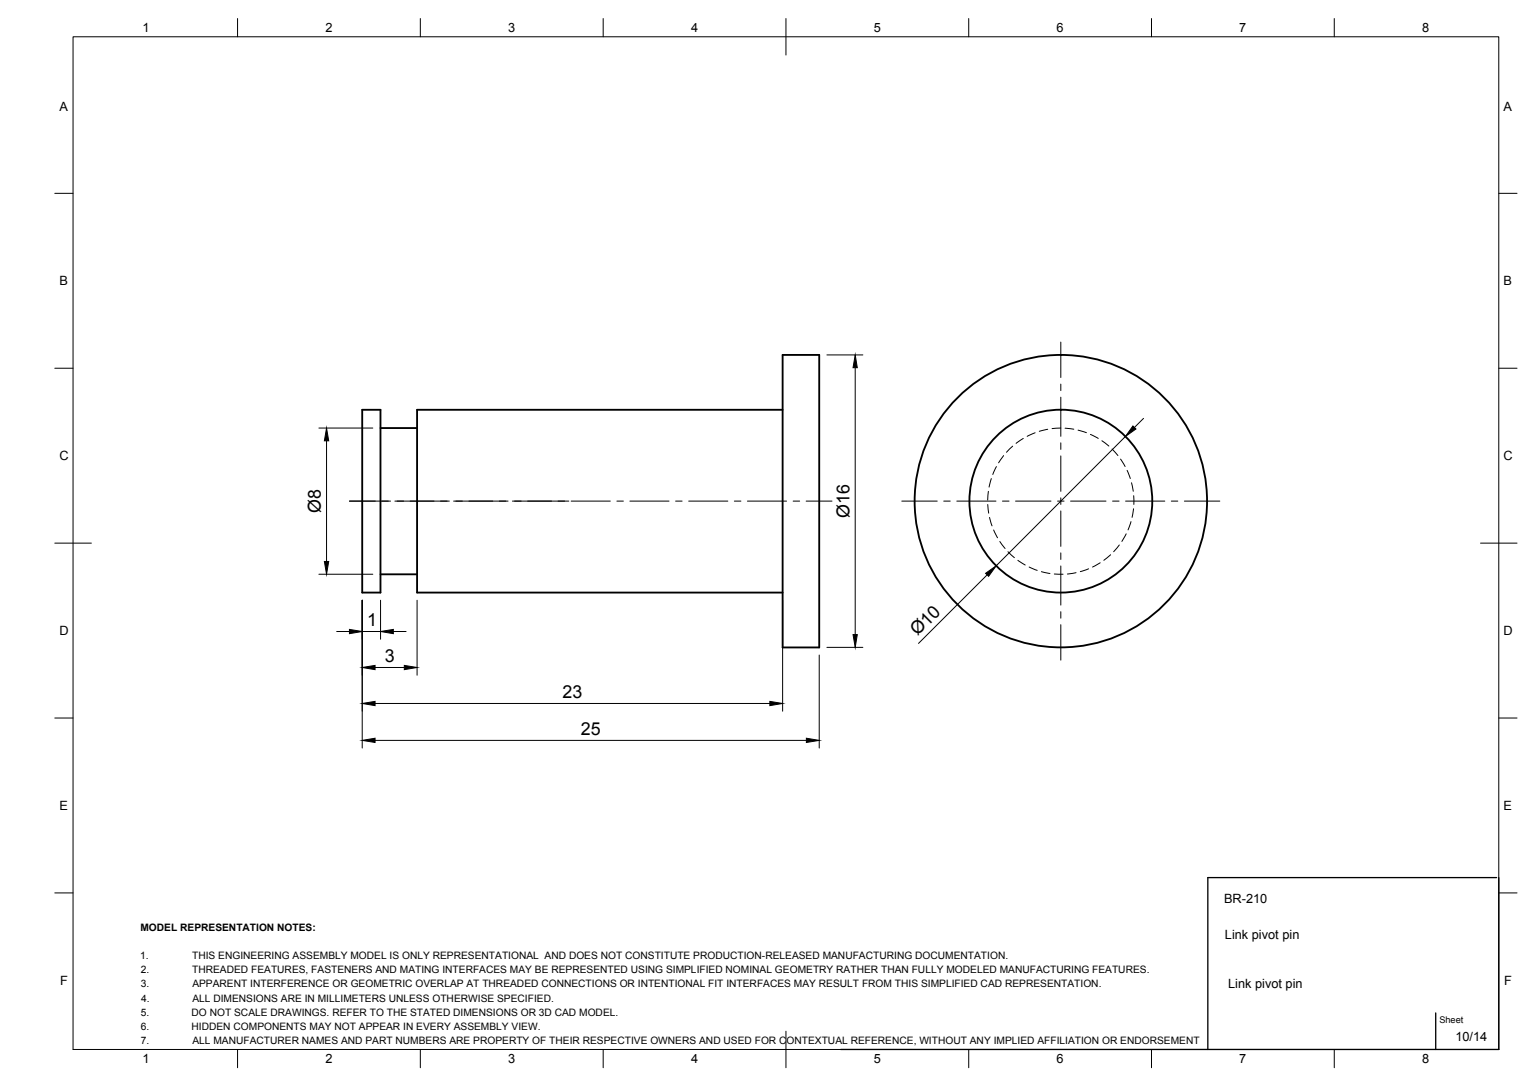
ISO-10303-21;
HEADER;
/* Generated by software containing ST-Developer
 * from STEP Tools, Inc. (www.steptools.com) 
 */

FILE_DESCRIPTION(
/* description */ ('Independent 1:2 reduction pantograph. 120 mm parallelogram sides; fix
ed fulcrum on the extension of a 240 mm link. Drawing point halfway al
ong its link, so its XY displacement is one half of the tracing point.
 Replaceable pivot bushes and retained pins. Calibration and productio
n accuracy unassigned.'),
/* implementation_level */ '2;1');

FILE_NAME(
/* name */ 'Link pivot pin.step',
/* time_stamp */ '2026-11-07T22:11:57-08:00',
/* author */ (''),
/* organization */ (''),
/* preprocessor_version */ 'ST-DEVELOPER v20.2',
/* originating_system */ 'Autodesk Translation Framework v15.17.0.0',
/* authorisation */ '');

FILE_SCHEMA (('AUTOMOTIVE_DESIGN { 1 0 10303 214 3 1 1 }'));
ENDSEC;

DATA;
#10=MECHANICAL_DESIGN_GEOMETRIC_PRESENTATION_REPRESENTATION('',(#195),#2926);
#169=SHAPE_REPRESENTATION_RELATIONSHIP('SRR','None',#3006,#182);
#182=ADVANCED_BREP_SHAPE_REPRESENTATION('',(#208),#2922);
#195=STYLED_ITEM('',(#3075),#208);
#208=MANIFOLD_SOLID_BREP('Body1',#1550);
#253=FACE_BOUND('',#510,.T.);
#254=FACE_BOUND('',#512,.T.);
#255=FACE_BOUND('',#515,.T.);
#293=PLANE('',#1852);
#294=PLANE('',#1854);
#295=PLANE('',#1858);
#296=PLANE('',#1863);
#297=PLANE('',#1865);
#375=FACE_OUTER_BOUND('',#508,.T.);
#376=FACE_OUTER_BOUND('',#509,.T.);
#377=FACE_OUTER_BOUND('',#511,.T.);
#378=FACE_OUTER_BOUND('',#513,.T.);
#379=FACE_OUTER_BOUND('',#514,.T.);
#380=FACE_OUTER_BOUND('',#516,.T.);
#381=FACE_OUTER_BOUND('',#517,.T.);
#382=FACE_OUTER_BOUND('',#518,.T.);
#383=FACE_OUTER_BOUND('',#519,.T.);
#508=EDGE_LOOP('',(#1337,#1338,#1339,#1340));
#509=EDGE_LOOP('',(#1341));
#510=EDGE_LOOP('',(#1342));
#511=EDGE_LOOP('',(#1343));
#512=EDGE_LOOP('',(#1344));
#513=EDGE_LOOP('',(#1345,#1346,#1347,#1348));
#514=EDGE_LOOP('',(#1349));
#515=EDGE_LOOP('',(#1350));
#516=EDGE_LOOP('',(#1351,#1352,#1353,#1354));
#517=EDGE_LOOP('',(#1355));
#518=EDGE_LOOP('',(#1356,#1357,#1358,#1359));
#519=EDGE_LOOP('',(#1360));
#600=LINE('',#2782,#681);
#601=LINE('',#2793,#682);
#602=LINE('',#2801,#683);
#603=LINE('',#2805,#684);
#681=VECTOR('',#2300,4.);
#682=VECTOR('',#2315,5.);
#683=VECTOR('',#2324,8.);
#684=VECTOR('',#2331,5.);
#767=CIRCLE('',#1850,4.);
#768=CIRCLE('',#1851,4.);
#769=CIRCLE('',#1853,5.);
#770=CIRCLE('',#1855,5.);
#771=CIRCLE('',#1857,5.);
#772=CIRCLE('',#1859,8.);
#773=CIRCLE('',#1860,5.);
#774=CIRCLE('',#1862,8.);
#875=VERTEX_POINT('',#2779);
#876=VERTEX_POINT('',#2781);
#877=VERTEX_POINT('',#2785);
#878=VERTEX_POINT('',#2788);
#879=VERTEX_POINT('',#2791);
#880=VERTEX_POINT('',#2795);
#881=VERTEX_POINT('',#2797);
#882=VERTEX_POINT('',#2800);
#1033=EDGE_CURVE('',#875,#875,#767,.T.);
#1034=EDGE_CURVE('',#875,#876,#600,.T.);
#1035=EDGE_CURVE('',#876,#876,#768,.T.);
#1036=EDGE_CURVE('',#877,#877,#769,.T.);
#1037=EDGE_CURVE('',#878,#878,#770,.T.);
#1038=EDGE_CURVE('',#879,#879,#771,.T.);
#1039=EDGE_CURVE('',#879,#878,#601,.T.);
#1040=EDGE_CURVE('',#880,#880,#772,.T.);
#1041=EDGE_CURVE('',#881,#881,#773,.T.);
#1042=EDGE_CURVE('',#880,#882,#602,.T.);
#1043=EDGE_CURVE('',#882,#882,#774,.T.);
#1044=EDGE_CURVE('',#877,#881,#603,.T.);
#1337=ORIENTED_EDGE('',*,*,#1033,.T.);
#1338=ORIENTED_EDGE('',*,*,#1034,.T.);
#1339=ORIENTED_EDGE('',*,*,#1035,.F.);
#1340=ORIENTED_EDGE('',*,*,#1034,.F.);
#1341=ORIENTED_EDGE('',*,*,#1036,.F.);
#1342=ORIENTED_EDGE('',*,*,#1033,.F.);
#1343=ORIENTED_EDGE('',*,*,#1037,.F.);
#1344=ORIENTED_EDGE('',*,*,#1035,.T.);
#1345=ORIENTED_EDGE('',*,*,#1038,.F.);
#1346=ORIENTED_EDGE('',*,*,#1039,.T.);
#1347=ORIENTED_EDGE('',*,*,#1037,.T.);
#1348=ORIENTED_EDGE('',*,*,#1039,.F.);
#1349=ORIENTED_EDGE('',*,*,#1040,.T.);
#1350=ORIENTED_EDGE('',*,*,#1041,.F.);
#1351=ORIENTED_EDGE('',*,*,#1040,.F.);
#1352=ORIENTED_EDGE('',*,*,#1042,.T.);
#1353=ORIENTED_EDGE('',*,*,#1043,.T.);
#1354=ORIENTED_EDGE('',*,*,#1042,.F.);
#1355=ORIENTED_EDGE('',*,*,#1043,.F.);
#1356=ORIENTED_EDGE('',*,*,#1036,.T.);
#1357=ORIENTED_EDGE('',*,*,#1044,.T.);
#1358=ORIENTED_EDGE('',*,*,#1041,.T.);
#1359=ORIENTED_EDGE('',*,*,#1044,.F.);
#1360=ORIENTED_EDGE('',*,*,#1038,.T.);
#1440=CYLINDRICAL_SURFACE('',#1849,4.);
#1441=CYLINDRICAL_SURFACE('',#1856,5.);
#1442=CYLINDRICAL_SURFACE('',#1861,8.);
#1443=CYLINDRICAL_SURFACE('',#1864,5.);
#1519=ADVANCED_FACE('',(#375),#1440,.T.);
#1520=ADVANCED_FACE('',(#376,#253),#293,.F.);
#1521=ADVANCED_FACE('',(#377,#254),#294,.F.);
#1522=ADVANCED_FACE('',(#378),#1441,.T.);
#1523=ADVANCED_FACE('',(#379,#255),#295,.T.);
#1524=ADVANCED_FACE('',(#380),#1442,.T.);
#1525=ADVANCED_FACE('',(#381),#296,.F.);
#1526=ADVANCED_FACE('',(#382),#1443,.T.);
#1527=ADVANCED_FACE('',(#383),#297,.T.);
#1550=CLOSED_SHELL('',(#1519,#1520,#1521,#1522,#1523,#1524,#1525,#1526,
#1527));
#1848=AXIS2_PLACEMENT_3D('',#2777,#2294,#2295);
#1849=AXIS2_PLACEMENT_3D('',#2778,#2296,#2297);
#1850=AXIS2_PLACEMENT_3D('',#2780,#2298,#2299);
#1851=AXIS2_PLACEMENT_3D('',#2783,#2301,#2302);
#1852=AXIS2_PLACEMENT_3D('',#2784,#2303,#2304);
#1853=AXIS2_PLACEMENT_3D('',#2786,#2305,#2306);
#1854=AXIS2_PLACEMENT_3D('',#2787,#2307,#2308);
#1855=AXIS2_PLACEMENT_3D('',#2789,#2309,#2310);
#1856=AXIS2_PLACEMENT_3D('',#2790,#2311,#2312);
#1857=AXIS2_PLACEMENT_3D('',#2792,#2313,#2314);
#1858=AXIS2_PLACEMENT_3D('',#2794,#2316,#2317);
#1859=AXIS2_PLACEMENT_3D('',#2796,#2318,#2319);
#1860=AXIS2_PLACEMENT_3D('',#2798,#2320,#2321);
#1861=AXIS2_PLACEMENT_3D('',#2799,#2322,#2323);
#1862=AXIS2_PLACEMENT_3D('',#2802,#2325,#2326);
#1863=AXIS2_PLACEMENT_3D('',#2803,#2327,#2328);
#1864=AXIS2_PLACEMENT_3D('',#2804,#2329,#2330);
#1865=AXIS2_PLACEMENT_3D('',#2806,#2332,#2333);
#2294=DIRECTION('axis',(0.,0.,1.));
#2295=DIRECTION('refdir',(1.,0.,0.));
#2296=DIRECTION('center_axis',(0.,0.,1.));
#2297=DIRECTION('ref_axis',(1.,0.,0.));
#2298=DIRECTION('center_axis',(0.,0.,1.));
#2299=DIRECTION('ref_axis',(1.,0.,0.));
#2300=DIRECTION('',(0.,0.,1.));
#2301=DIRECTION('center_axis',(0.,0.,1.));
#2302=DIRECTION('ref_axis',(1.,0.,0.));
#2303=DIRECTION('center_axis',(0.,0.,-1.));
#2304=DIRECTION('ref_axis',(-1.,0.,0.));
#2305=DIRECTION('center_axis',(0.,0.,-1.));
#2306=DIRECTION('ref_axis',(1.,0.,0.));
#2307=DIRECTION('center_axis',(0.,0.,1.));
#2308=DIRECTION('ref_axis',(1.,0.,0.));
#2309=DIRECTION('center_axis',(0.,0.,1.));
#2310=DIRECTION('ref_axis',(1.,0.,0.));
#2311=DIRECTION('center_axis',(0.,0.,1.));
#2312=DIRECTION('ref_axis',(1.,0.,0.));
#2313=DIRECTION('center_axis',(0.,0.,1.));
#2314=DIRECTION('ref_axis',(1.,0.,0.));
#2315=DIRECTION('',(0.,0.,-1.));
#2316=DIRECTION('center_axis',(0.,0.,1.));
#2317=DIRECTION('ref_axis',(1.,0.,0.));
#2318=DIRECTION('center_axis',(0.,0.,1.));
#2319=DIRECTION('ref_axis',(1.,0.,0.));
#2320=DIRECTION('center_axis',(0.,0.,1.));
#2321=DIRECTION('ref_axis',(1.,0.,0.));
#2322=DIRECTION('center_axis',(0.,0.,1.));
#2323=DIRECTION('ref_axis',(1.,0.,0.));
#2324=DIRECTION('',(0.,0.,-1.));
#2325=DIRECTION('center_axis',(0.,0.,1.));
#2326=DIRECTION('ref_axis',(1.,0.,0.));
#2327=DIRECTION('center_axis',(0.,0.,1.));
#2328=DIRECTION('ref_axis',(1.,0.,0.));
#2329=DIRECTION('center_axis',(0.,0.,1.));
#2330=DIRECTION('ref_axis',(1.,0.,0.));
#2331=DIRECTION('',(0.,0.,-1.));
#2332=DIRECTION('center_axis',(0.,0.,1.));
#2333=DIRECTION('ref_axis',(1.,0.,0.));
#2777=CARTESIAN_POINT('',(0.,0.,0.));
#2778=CARTESIAN_POINT('Origin',(0.,0.,21.));
#2779=CARTESIAN_POINT('',(-4.,-4.89858719658941E-16,20.));
#2780=CARTESIAN_POINT('Origin',(0.,0.,20.));
#2781=CARTESIAN_POINT('',(-4.,-4.89858719658941E-16,22.));
#2782=CARTESIAN_POINT('',(-4.,-4.89858719658941E-16,21.));
#2783=CARTESIAN_POINT('Origin',(0.,0.,22.));
#2784=CARTESIAN_POINT('Origin',(8.,0.,20.));
#2785=CARTESIAN_POINT('',(-5.,6.12323399573677E-16,20.));
#2786=CARTESIAN_POINT('Origin',(0.,0.,20.));
#2787=CARTESIAN_POINT('Origin',(4.,0.,22.));
#2788=CARTESIAN_POINT('',(-5.,-6.12323399573677E-16,22.));
#2789=CARTESIAN_POINT('Origin',(0.,0.,22.));
#2790=CARTESIAN_POINT('Origin',(0.,0.,0.));
#2791=CARTESIAN_POINT('',(-5.,-6.12323399573677E-16,23.));
#2792=CARTESIAN_POINT('Origin',(0.,0.,23.));
#2793=CARTESIAN_POINT('',(-5.,-6.12323399573677E-16,0.));
#2794=CARTESIAN_POINT('Origin',(0.,0.,0.));
#2795=CARTESIAN_POINT('',(-8.,-9.79717439317883E-16,0.));
#2796=CARTESIAN_POINT('Origin',(0.,0.,0.));
#2797=CARTESIAN_POINT('',(-5.,-6.12323399573677E-16,0.));
#2798=CARTESIAN_POINT('Origin',(0.,0.,0.));
#2799=CARTESIAN_POINT('Origin',(0.,0.,-2.));
#2800=CARTESIAN_POINT('',(-8.,-9.79717439317883E-16,-2.));
#2801=CARTESIAN_POINT('',(-8.,-9.79717439317883E-16,-2.));
#2802=CARTESIAN_POINT('Origin',(0.,0.,-2.));
#2803=CARTESIAN_POINT('Origin',(0.,0.,-2.));
#2804=CARTESIAN_POINT('Origin',(0.,0.,0.));
#2805=CARTESIAN_POINT('',(-5.,-6.12323399573677E-16,0.));
#2806=CARTESIAN_POINT('Origin',(0.,0.,23.));
#2907=UNCERTAINTY_MEASURE_WITH_UNIT(LENGTH_MEASURE(0.01),#2927,
'DISTANCE_ACCURACY_VALUE',
'Maximum model space distance between geometric entities at asserted c
onnectivities');
#2911=UNCERTAINTY_MEASURE_WITH_UNIT(LENGTH_MEASURE(0.01),#2927,
'DISTANCE_ACCURACY_VALUE',
'Maximum model space distance between geometric entities at asserted c
onnectivities');
#2922=(
GEOMETRIC_REPRESENTATION_CONTEXT(3)
GLOBAL_UNCERTAINTY_ASSIGNED_CONTEXT((#2907))
GLOBAL_UNIT_ASSIGNED_CONTEXT((#2927,#2929,#2930))
REPRESENTATION_CONTEXT('','3D')
);
#2926=(
GEOMETRIC_REPRESENTATION_CONTEXT(3)
GLOBAL_UNCERTAINTY_ASSIGNED_CONTEXT((#2911))
GLOBAL_UNIT_ASSIGNED_CONTEXT((#2927,#2929,#2930))
REPRESENTATION_CONTEXT('','3D')
);
#2927=(
LENGTH_UNIT()
NAMED_UNIT(*)
SI_UNIT(.MILLI.,.METRE.)
);
#2929=(
NAMED_UNIT(*)
PLANE_ANGLE_UNIT()
SI_UNIT($,.RADIAN.)
);
#2930=(
NAMED_UNIT(*)
SI_UNIT($,.STERADIAN.)
SOLID_ANGLE_UNIT()
);
#2941=SHAPE_DEFINITION_REPRESENTATION(#2955,#3006);
#2955=PRODUCT_DEFINITION_SHAPE('',$,#3021);
#3006=SHAPE_REPRESENTATION('',(#1848),#2922);
#3010=PRODUCT_DEFINITION_CONTEXT('part definition',#3054,'design');
#3021=PRODUCT_DEFINITION('Link pivot pin','Link pivot pin',#3035,#3010);
#3035=PRODUCT_DEFINITION_FORMATION('',$,#3066);
#3054=APPLICATION_CONTEXT(
'Core Data for Automotive Mechanical Design Process');
#3055=PRODUCT_CONTEXT('part definition',#3054,'mechanical');
#3066=PRODUCT('Link pivot pin','Link pivot pin',$,(#3055));
#3075=PRESENTATION_STYLE_ASSIGNMENT((#3087));
#3087=SURFACE_STYLE_USAGE(.BOTH.,#3099);
#3099=SURFACE_SIDE_STYLE('',(#3111));
#3111=SURFACE_STYLE_FILL_AREA(#3123);
#3123=FILL_AREA_STYLE('Pivot gray',(#3135));
#3135=FILL_AREA_STYLE_COLOUR('Pivot gray',#3147);
#3147=COLOUR_RGB('Pivot gray',0.407843137254902,0.447058823529412,0.498039215686275);
ENDSEC;
END-ISO-10303-21;
